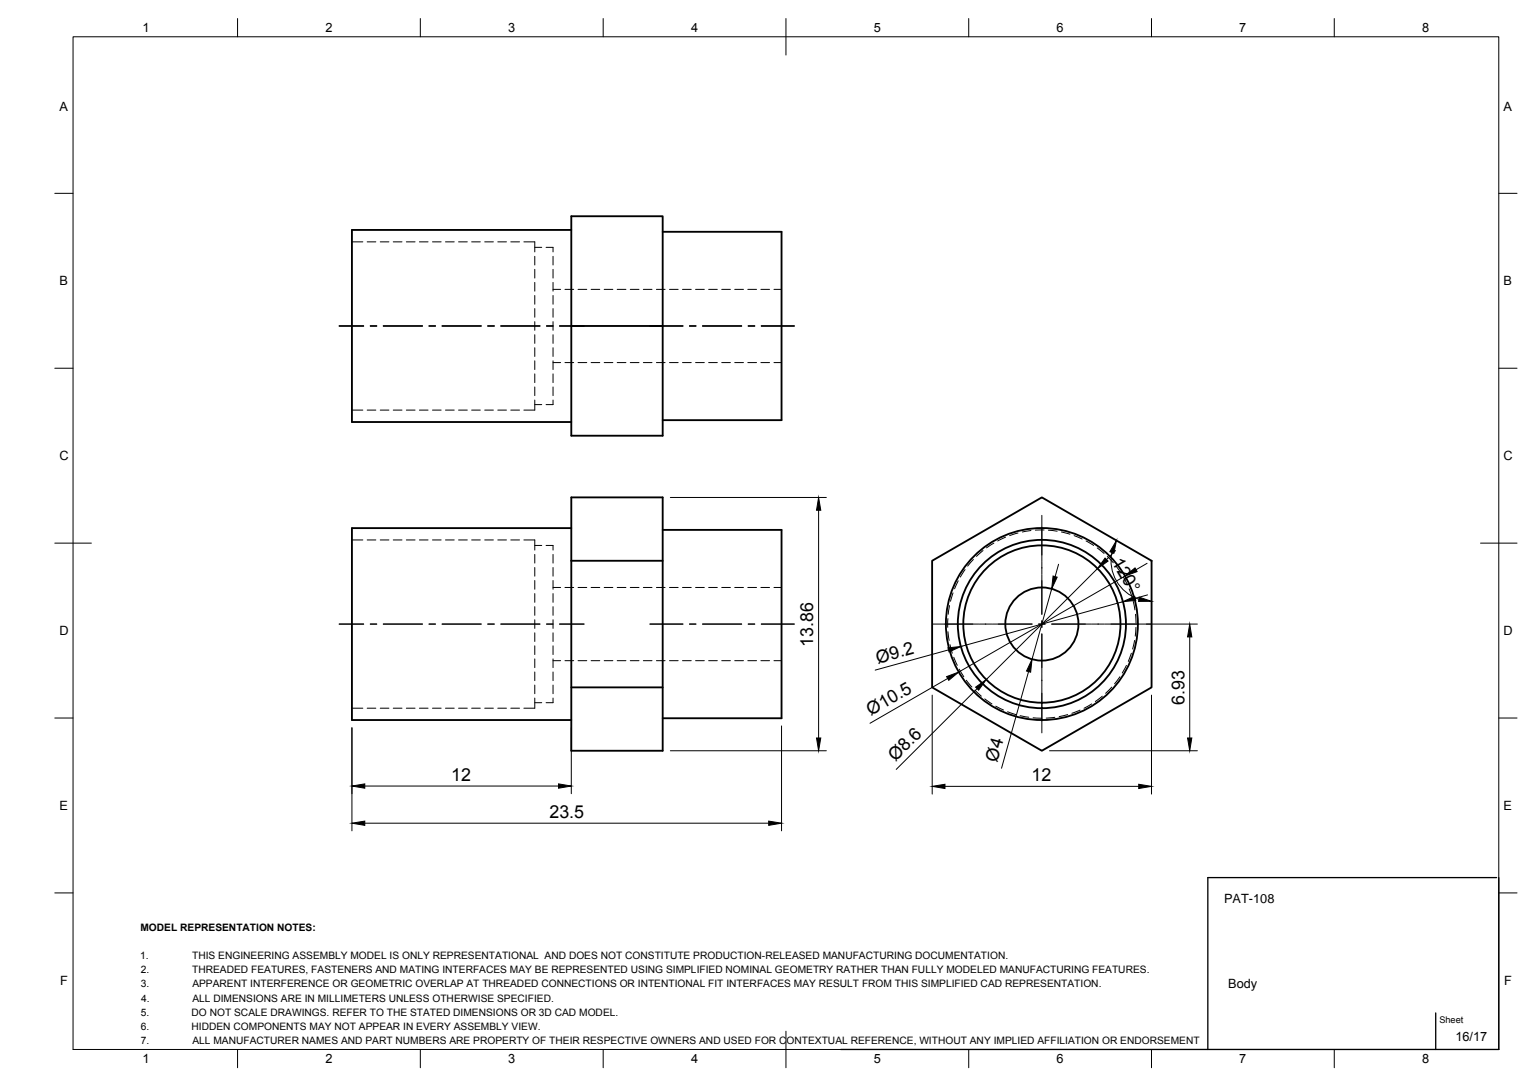
ISO-10303-21;
HEADER;
/* Generated by software containing ST-Developer
 * from STEP Tools, Inc. (www.steptools.com) 
 */

FILE_DESCRIPTION(
/* description */ ('Sub-base valve envelopes and connections'),
/* implementation_level */ '2;1');

FILE_NAME(
/* name */ 'Body.step',
/* time_stamp */ '2026-10-29T15:55:44-07:00',
/* author */ (''),
/* organization */ (''),
/* preprocessor_version */ 'ST-DEVELOPER v20.2',
/* originating_system */ 'Autodesk Translation Framework v15.17.0.0',
/* authorisation */ '');

FILE_SCHEMA (('AUTOMOTIVE_DESIGN { 1 0 10303 214 3 1 1 }'));
ENDSEC;

DATA;
#10=MECHANICAL_DESIGN_GEOMETRIC_PRESENTATION_REPRESENTATION('',(#128),#6113);
#104=SHAPE_REPRESENTATION_RELATIONSHIP('SRR','None',#6179,#116);
#116=ADVANCED_BREP_SHAPE_REPRESENTATION('',(#140),#6110);
#128=STYLED_ITEM('',(#6294),#140);
#140=MANIFOLD_SOLID_BREP('Body1',#3367);
#249=FACE_BOUND('',#853,.T.);
#250=FACE_BOUND('',#855,.T.);
#251=FACE_BOUND('',#857,.T.);
#252=FACE_BOUND('',#865,.T.);
#253=FACE_BOUND('',#868,.T.);
#254=FACE_BOUND('',#872,.T.);
#360=PLANE('',#3823);
#361=PLANE('',#3825);
#362=PLANE('',#3827);
#363=PLANE('',#3829);
#364=PLANE('',#3830);
#365=PLANE('',#3831);
#366=PLANE('',#3832);
#367=PLANE('',#3833);
#368=PLANE('',#3834);
#369=PLANE('',#3835);
#370=PLANE('',#3839);
#371=PLANE('',#3844);
#545=FACE_OUTER_BOUND('',#851,.T.);
#546=FACE_OUTER_BOUND('',#852,.T.);
#547=FACE_OUTER_BOUND('',#854,.T.);
#548=FACE_OUTER_BOUND('',#856,.T.);
#549=FACE_OUTER_BOUND('',#858,.T.);
#550=FACE_OUTER_BOUND('',#859,.T.);
#551=FACE_OUTER_BOUND('',#860,.T.);
#552=FACE_OUTER_BOUND('',#861,.T.);
#553=FACE_OUTER_BOUND('',#862,.T.);
#554=FACE_OUTER_BOUND('',#863,.T.);
#555=FACE_OUTER_BOUND('',#864,.T.);
#556=FACE_OUTER_BOUND('',#866,.T.);
#557=FACE_OUTER_BOUND('',#867,.T.);
#558=FACE_OUTER_BOUND('',#869,.T.);
#559=FACE_OUTER_BOUND('',#870,.T.);
#560=FACE_OUTER_BOUND('',#871,.T.);
#561=FACE_OUTER_BOUND('',#873,.T.);
#851=EDGE_LOOP('',(#2927,#2928,#2929,#2930));
#852=EDGE_LOOP('',(#2931));
#853=EDGE_LOOP('',(#2932));
#854=EDGE_LOOP('',(#2933,#2934,#2935,#2936,#2937,#2938));
#855=EDGE_LOOP('',(#2939));
#856=EDGE_LOOP('',(#2940,#2941,#2942,#2943,#2944,#2945));
#857=EDGE_LOOP('',(#2946));
#858=EDGE_LOOP('',(#2947,#2948,#2949,#2950));
#859=EDGE_LOOP('',(#2951,#2952,#2953,#2954));
#860=EDGE_LOOP('',(#2955,#2956,#2957,#2958));
#861=EDGE_LOOP('',(#2959,#2960,#2961,#2962));
#862=EDGE_LOOP('',(#2963,#2964,#2965,#2966));
#863=EDGE_LOOP('',(#2967,#2968,#2969,#2970));
#864=EDGE_LOOP('',(#2971));
#865=EDGE_LOOP('',(#2972));
#866=EDGE_LOOP('',(#2973,#2974,#2975,#2976));
#867=EDGE_LOOP('',(#2977));
#868=EDGE_LOOP('',(#2978));
#869=EDGE_LOOP('',(#2979,#2980,#2981,#2982));
#870=EDGE_LOOP('',(#2983,#2984,#2985,#2986));
#871=EDGE_LOOP('',(#2987));
#872=EDGE_LOOP('',(#2988));
#873=EDGE_LOOP('',(#2989,#2990,#2991,#2992));
#1085=LINE('',#5903,#1319);
#1086=LINE('',#5911,#1320);
#1087=LINE('',#5913,#1321);
#1088=LINE('',#5915,#1322);
#1089=LINE('',#5917,#1323);
#1090=LINE('',#5919,#1324);
#1091=LINE('',#5920,#1325);
#1092=LINE('',#5926,#1326);
#1093=LINE('',#5928,#1327);
#1094=LINE('',#5930,#1328);
#1095=LINE('',#5932,#1329);
#1096=LINE('',#5934,#1330);
#1097=LINE('',#5935,#1331);
#1098=LINE('',#5939,#1332);
#1099=LINE('',#5940,#1333);
#1100=LINE('',#5942,#1334);
#1101=LINE('',#5944,#1335);
#1102=LINE('',#5946,#1336);
#1103=LINE('',#5948,#1337);
#1104=LINE('',#5955,#1338);
#1105=LINE('',#5961,#1339);
#1106=LINE('',#5965,#1340);
#1107=LINE('',#5970,#1341);
#1319=VECTOR('',#4725,0.43);
#1320=VECTOR('',#4734,1.);
#1321=VECTOR('',#4735,1.);
#1322=VECTOR('',#4736,1.);
#1323=VECTOR('',#4737,1.);
#1324=VECTOR('',#4738,1.);
#1325=VECTOR('',#4739,1.);
#1326=VECTOR('',#4744,1.);
#1327=VECTOR('',#4745,1.);
#1328=VECTOR('',#4746,1.);
#1329=VECTOR('',#4747,1.);
#1330=VECTOR('',#4748,1.);
#1331=VECTOR('',#4749,1.);
#1332=VECTOR('',#4754,1.);
#1333=VECTOR('',#4755,1.);
#1334=VECTOR('',#4758,1.);
#1335=VECTOR('',#4761,1.);
#1336=VECTOR('',#4764,1.);
#1337=VECTOR('',#4767,1.);
#1338=VECTOR('',#4776,0.46);
#1339=VECTOR('',#4785,0.525);
#1340=VECTOR('',#4790,0.515);
#1341=VECTOR('',#4797,0.2);
#1513=CIRCLE('',#3821,0.43);
#1514=CIRCLE('',#3822,0.43);
#1515=CIRCLE('',#3824,0.2);
#1516=CIRCLE('',#3826,0.525);
#1517=CIRCLE('',#3828,0.515);
#1518=CIRCLE('',#3836,0.46);
#1519=CIRCLE('',#3838,0.46);
#1520=CIRCLE('',#3840,0.525);
#1521=CIRCLE('',#3843,0.515);
#1522=CIRCLE('',#3845,0.2);
#1767=VERTEX_POINT('',#5900);
#1768=VERTEX_POINT('',#5902);
#1769=VERTEX_POINT('',#5906);
#1770=VERTEX_POINT('',#5909);
#1771=VERTEX_POINT('',#5910);
#1772=VERTEX_POINT('',#5912);
#1773=VERTEX_POINT('',#5914);
#1774=VERTEX_POINT('',#5916);
#1775=VERTEX_POINT('',#5918);
#1776=VERTEX_POINT('',#5921);
#1777=VERTEX_POINT('',#5924);
#1778=VERTEX_POINT('',#5925);
#1779=VERTEX_POINT('',#5927);
#1780=VERTEX_POINT('',#5929);
#1781=VERTEX_POINT('',#5931);
#1782=VERTEX_POINT('',#5933);
#1783=VERTEX_POINT('',#5936);
#1784=VERTEX_POINT('',#5951);
#1785=VERTEX_POINT('',#5954);
#1786=VERTEX_POINT('',#5958);
#1787=VERTEX_POINT('',#5963);
#1788=VERTEX_POINT('',#5967);
#2161=EDGE_CURVE('',#1767,#1767,#1513,.T.);
#2162=EDGE_CURVE('',#1767,#1768,#1085,.T.);
#2163=EDGE_CURVE('',#1768,#1768,#1514,.T.);
#2164=EDGE_CURVE('',#1769,#1769,#1515,.T.);
#2165=EDGE_CURVE('',#1770,#1771,#1086,.T.);
#2166=EDGE_CURVE('',#1771,#1772,#1087,.T.);
#2167=EDGE_CURVE('',#1772,#1773,#1088,.T.);
#2168=EDGE_CURVE('',#1773,#1774,#1089,.T.);
#2169=EDGE_CURVE('',#1774,#1775,#1090,.T.);
#2170=EDGE_CURVE('',#1775,#1770,#1091,.T.);
#2171=EDGE_CURVE('',#1776,#1776,#1516,.T.);
#2172=EDGE_CURVE('',#1777,#1778,#1092,.T.);
#2173=EDGE_CURVE('',#1779,#1777,#1093,.T.);
#2174=EDGE_CURVE('',#1780,#1779,#1094,.T.);
#2175=EDGE_CURVE('',#1781,#1780,#1095,.T.);
#2176=EDGE_CURVE('',#1782,#1781,#1096,.T.);
#2177=EDGE_CURVE('',#1778,#1782,#1097,.T.);
#2178=EDGE_CURVE('',#1783,#1783,#1517,.T.);
#2179=EDGE_CURVE('',#1777,#1770,#1098,.T.);
#2180=EDGE_CURVE('',#1779,#1775,#1099,.T.);
#2181=EDGE_CURVE('',#1780,#1774,#1100,.T.);
#2182=EDGE_CURVE('',#1781,#1773,#1101,.T.);
#2183=EDGE_CURVE('',#1782,#1772,#1102,.T.);
#2184=EDGE_CURVE('',#1778,#1771,#1103,.T.);
#2185=EDGE_CURVE('',#1784,#1784,#1518,.T.);
#2186=EDGE_CURVE('',#1784,#1785,#1104,.T.);
#2187=EDGE_CURVE('',#1785,#1785,#1519,.T.);
#2188=EDGE_CURVE('',#1786,#1786,#1520,.T.);
#2189=EDGE_CURVE('',#1776,#1786,#1105,.T.);
#2190=EDGE_CURVE('',#1787,#1787,#1521,.T.);
#2191=EDGE_CURVE('',#1787,#1783,#1106,.T.);
#2192=EDGE_CURVE('',#1788,#1788,#1522,.T.);
#2193=EDGE_CURVE('',#1788,#1769,#1107,.T.);
#2927=ORIENTED_EDGE('',*,*,#2161,.F.);
#2928=ORIENTED_EDGE('',*,*,#2162,.T.);
#2929=ORIENTED_EDGE('',*,*,#2163,.F.);
#2930=ORIENTED_EDGE('',*,*,#2162,.F.);
#2931=ORIENTED_EDGE('',*,*,#2161,.T.);
#2932=ORIENTED_EDGE('',*,*,#2164,.F.);
#2933=ORIENTED_EDGE('',*,*,#2165,.T.);
#2934=ORIENTED_EDGE('',*,*,#2166,.T.);
#2935=ORIENTED_EDGE('',*,*,#2167,.T.);
#2936=ORIENTED_EDGE('',*,*,#2168,.T.);
#2937=ORIENTED_EDGE('',*,*,#2169,.T.);
#2938=ORIENTED_EDGE('',*,*,#2170,.T.);
#2939=ORIENTED_EDGE('',*,*,#2171,.T.);
#2940=ORIENTED_EDGE('',*,*,#2172,.F.);
#2941=ORIENTED_EDGE('',*,*,#2173,.F.);
#2942=ORIENTED_EDGE('',*,*,#2174,.F.);
#2943=ORIENTED_EDGE('',*,*,#2175,.F.);
#2944=ORIENTED_EDGE('',*,*,#2176,.F.);
#2945=ORIENTED_EDGE('',*,*,#2177,.F.);
#2946=ORIENTED_EDGE('',*,*,#2178,.F.);
#2947=ORIENTED_EDGE('',*,*,#2173,.T.);
#2948=ORIENTED_EDGE('',*,*,#2179,.T.);
#2949=ORIENTED_EDGE('',*,*,#2170,.F.);
#2950=ORIENTED_EDGE('',*,*,#2180,.F.);
#2951=ORIENTED_EDGE('',*,*,#2174,.T.);
#2952=ORIENTED_EDGE('',*,*,#2180,.T.);
#2953=ORIENTED_EDGE('',*,*,#2169,.F.);
#2954=ORIENTED_EDGE('',*,*,#2181,.F.);
#2955=ORIENTED_EDGE('',*,*,#2175,.T.);
#2956=ORIENTED_EDGE('',*,*,#2181,.T.);
#2957=ORIENTED_EDGE('',*,*,#2168,.F.);
#2958=ORIENTED_EDGE('',*,*,#2182,.F.);
#2959=ORIENTED_EDGE('',*,*,#2176,.T.);
#2960=ORIENTED_EDGE('',*,*,#2182,.T.);
#2961=ORIENTED_EDGE('',*,*,#2167,.F.);
#2962=ORIENTED_EDGE('',*,*,#2183,.F.);
#2963=ORIENTED_EDGE('',*,*,#2177,.T.);
#2964=ORIENTED_EDGE('',*,*,#2183,.T.);
#2965=ORIENTED_EDGE('',*,*,#2166,.F.);
#2966=ORIENTED_EDGE('',*,*,#2184,.F.);
#2967=ORIENTED_EDGE('',*,*,#2172,.T.);
#2968=ORIENTED_EDGE('',*,*,#2184,.T.);
#2969=ORIENTED_EDGE('',*,*,#2165,.F.);
#2970=ORIENTED_EDGE('',*,*,#2179,.F.);
#2971=ORIENTED_EDGE('',*,*,#2185,.F.);
#2972=ORIENTED_EDGE('',*,*,#2163,.T.);
#2973=ORIENTED_EDGE('',*,*,#2185,.T.);
#2974=ORIENTED_EDGE('',*,*,#2186,.T.);
#2975=ORIENTED_EDGE('',*,*,#2187,.F.);
#2976=ORIENTED_EDGE('',*,*,#2186,.F.);
#2977=ORIENTED_EDGE('',*,*,#2188,.F.);
#2978=ORIENTED_EDGE('',*,*,#2187,.T.);
#2979=ORIENTED_EDGE('',*,*,#2171,.F.);
#2980=ORIENTED_EDGE('',*,*,#2189,.T.);
#2981=ORIENTED_EDGE('',*,*,#2188,.T.);
#2982=ORIENTED_EDGE('',*,*,#2189,.F.);
#2983=ORIENTED_EDGE('',*,*,#2190,.F.);
#2984=ORIENTED_EDGE('',*,*,#2191,.T.);
#2985=ORIENTED_EDGE('',*,*,#2178,.T.);
#2986=ORIENTED_EDGE('',*,*,#2191,.F.);
#2987=ORIENTED_EDGE('',*,*,#2190,.T.);
#2988=ORIENTED_EDGE('',*,*,#2192,.F.);
#2989=ORIENTED_EDGE('',*,*,#2192,.T.);
#2990=ORIENTED_EDGE('',*,*,#2193,.T.);
#2991=ORIENTED_EDGE('',*,*,#2164,.T.);
#2992=ORIENTED_EDGE('',*,*,#2193,.F.);
#3149=CYLINDRICAL_SURFACE('',#3820,0.43);
#3150=CYLINDRICAL_SURFACE('',#3837,0.46);
#3151=CYLINDRICAL_SURFACE('',#3841,0.525);
#3152=CYLINDRICAL_SURFACE('',#3842,0.515);
#3153=CYLINDRICAL_SURFACE('',#3846,0.2);
#3318=ADVANCED_FACE('',(#545),#3149,.F.);
#3319=ADVANCED_FACE('',(#546,#249),#360,.T.);
#3320=ADVANCED_FACE('',(#547,#250),#361,.T.);
#3321=ADVANCED_FACE('',(#548,#251),#362,.F.);
#3322=ADVANCED_FACE('',(#549),#363,.T.);
#3323=ADVANCED_FACE('',(#550),#364,.T.);
#3324=ADVANCED_FACE('',(#551),#365,.T.);
#3325=ADVANCED_FACE('',(#552),#366,.T.);
#3326=ADVANCED_FACE('',(#553),#367,.T.);
#3327=ADVANCED_FACE('',(#554),#368,.T.);
#3328=ADVANCED_FACE('',(#555,#252),#369,.T.);
#3329=ADVANCED_FACE('',(#556),#3150,.F.);
#3330=ADVANCED_FACE('',(#557,#253),#370,.T.);
#3331=ADVANCED_FACE('',(#558),#3151,.T.);
#3332=ADVANCED_FACE('',(#559),#3152,.T.);
#3333=ADVANCED_FACE('',(#560,#254),#371,.T.);
#3334=ADVANCED_FACE('',(#561),#3153,.F.);
#3367=CLOSED_SHELL('',(#3318,#3319,#3320,#3321,#3322,#3323,#3324,#3325,
#3326,#3327,#3328,#3329,#3330,#3331,#3332,#3333,#3334));
#3819=AXIS2_PLACEMENT_3D('',#5898,#4719,#4720);
#3820=AXIS2_PLACEMENT_3D('',#5899,#4721,#4722);
#3821=AXIS2_PLACEMENT_3D('',#5901,#4723,#4724);
#3822=AXIS2_PLACEMENT_3D('',#5904,#4726,#4727);
#3823=AXIS2_PLACEMENT_3D('',#5905,#4728,#4729);
#3824=AXIS2_PLACEMENT_3D('',#5907,#4730,#4731);
#3825=AXIS2_PLACEMENT_3D('',#5908,#4732,#4733);
#3826=AXIS2_PLACEMENT_3D('',#5922,#4740,#4741);
#3827=AXIS2_PLACEMENT_3D('',#5923,#4742,#4743);
#3828=AXIS2_PLACEMENT_3D('',#5937,#4750,#4751);
#3829=AXIS2_PLACEMENT_3D('',#5938,#4752,#4753);
#3830=AXIS2_PLACEMENT_3D('',#5941,#4756,#4757);
#3831=AXIS2_PLACEMENT_3D('',#5943,#4759,#4760);
#3832=AXIS2_PLACEMENT_3D('',#5945,#4762,#4763);
#3833=AXIS2_PLACEMENT_3D('',#5947,#4765,#4766);
#3834=AXIS2_PLACEMENT_3D('',#5949,#4768,#4769);
#3835=AXIS2_PLACEMENT_3D('',#5950,#4770,#4771);
#3836=AXIS2_PLACEMENT_3D('',#5952,#4772,#4773);
#3837=AXIS2_PLACEMENT_3D('',#5953,#4774,#4775);
#3838=AXIS2_PLACEMENT_3D('',#5956,#4777,#4778);
#3839=AXIS2_PLACEMENT_3D('',#5957,#4779,#4780);
#3840=AXIS2_PLACEMENT_3D('',#5959,#4781,#4782);
#3841=AXIS2_PLACEMENT_3D('',#5960,#4783,#4784);
#3842=AXIS2_PLACEMENT_3D('',#5962,#4786,#4787);
#3843=AXIS2_PLACEMENT_3D('',#5964,#4788,#4789);
#3844=AXIS2_PLACEMENT_3D('',#5966,#4791,#4792);
#3845=AXIS2_PLACEMENT_3D('',#5968,#4793,#4794);
#3846=AXIS2_PLACEMENT_3D('',#5969,#4795,#4796);
#4719=DIRECTION('axis',(0.,0.,1.));
#4720=DIRECTION('refdir',(1.,0.,0.));
#4721=DIRECTION('center_axis',(0.,1.,0.));
#4722=DIRECTION('ref_axis',(1.,0.,0.));
#4723=DIRECTION('center_axis',(0.,1.,0.));
#4724=DIRECTION('ref_axis',(1.,0.,0.));
#4725=DIRECTION('',(0.,1.,0.));
#4726=DIRECTION('center_axis',(0.,-1.,0.));
#4727=DIRECTION('ref_axis',(1.,0.,0.));
#4728=DIRECTION('center_axis',(0.,1.,0.));
#4729=DIRECTION('ref_axis',(1.,0.,0.));
#4730=DIRECTION('center_axis',(0.,1.,0.));
#4731=DIRECTION('ref_axis',(1.,0.,0.));
#4732=DIRECTION('center_axis',(0.,1.,0.));
#4733=DIRECTION('ref_axis',(1.,0.,0.));
#4734=DIRECTION('',(0.5,0.,-0.866025403784439));
#4735=DIRECTION('',(-0.5,0.,-0.866025403784439));
#4736=DIRECTION('',(-1.,0.,-1.60246890531964E-16));
#4737=DIRECTION('',(-0.5,0.,0.866025403784439));
#4738=DIRECTION('',(0.5,0.,0.866025403784439));
#4739=DIRECTION('',(1.,0.,1.60246890531964E-16));
#4740=DIRECTION('center_axis',(0.,-1.,0.));
#4741=DIRECTION('ref_axis',(1.,0.,0.));
#4742=DIRECTION('center_axis',(0.,1.,0.));
#4743=DIRECTION('ref_axis',(1.,0.,0.));
#4744=DIRECTION('',(0.5,0.,-0.866025403784439));
#4745=DIRECTION('',(1.,0.,1.60246890531964E-16));
#4746=DIRECTION('',(0.5,0.,0.866025403784439));
#4747=DIRECTION('',(-0.5,0.,0.866025403784439));
#4748=DIRECTION('',(-1.,0.,-1.60246890531964E-16));
#4749=DIRECTION('',(-0.5,0.,-0.866025403784439));
#4750=DIRECTION('center_axis',(0.,-1.,0.));
#4751=DIRECTION('ref_axis',(1.,0.,0.));
#4752=DIRECTION('center_axis',(-1.60246890531964E-16,0.,1.));
#4753=DIRECTION('ref_axis',(1.,0.,1.60246890531964E-16));
#4754=DIRECTION('',(0.,1.,0.));
#4755=DIRECTION('',(0.,1.,0.));
#4756=DIRECTION('center_axis',(-0.866025403784439,0.,0.5));
#4757=DIRECTION('ref_axis',(0.5,0.,0.866025403784439));
#4758=DIRECTION('',(0.,1.,0.));
#4759=DIRECTION('center_axis',(-0.866025403784439,0.,-0.5));
#4760=DIRECTION('ref_axis',(-0.5,0.,0.866025403784439));
#4761=DIRECTION('',(0.,1.,0.));
#4762=DIRECTION('center_axis',(1.60246890531964E-16,0.,-1.));
#4763=DIRECTION('ref_axis',(-1.,0.,-1.60246890531964E-16));
#4764=DIRECTION('',(0.,1.,0.));
#4765=DIRECTION('center_axis',(0.866025403784439,0.,-0.5));
#4766=DIRECTION('ref_axis',(-0.5,0.,-0.866025403784439));
#4767=DIRECTION('',(0.,1.,0.));
#4768=DIRECTION('center_axis',(0.866025403784439,0.,0.5));
#4769=DIRECTION('ref_axis',(0.5,0.,-0.866025403784439));
#4770=DIRECTION('center_axis',(0.,1.,0.));
#4771=DIRECTION('ref_axis',(0.,0.,1.));
#4772=DIRECTION('center_axis',(0.,-1.,0.));
#4773=DIRECTION('ref_axis',(1.,0.,0.));
#4774=DIRECTION('center_axis',(0.,-1.,0.));
#4775=DIRECTION('ref_axis',(1.,0.,0.));
#4776=DIRECTION('',(0.,1.,0.));
#4777=DIRECTION('center_axis',(0.,-1.,0.));
#4778=DIRECTION('ref_axis',(1.,0.,0.));
#4779=DIRECTION('center_axis',(0.,1.,0.));
#4780=DIRECTION('ref_axis',(0.,0.,1.));
#4781=DIRECTION('center_axis',(0.,-1.,0.));
#4782=DIRECTION('ref_axis',(1.,0.,0.));
#4783=DIRECTION('center_axis',(0.,-1.,0.));
#4784=DIRECTION('ref_axis',(1.,0.,0.));
#4785=DIRECTION('',(0.,1.,0.));
#4786=DIRECTION('center_axis',(0.,-1.,0.));
#4787=DIRECTION('ref_axis',(1.,0.,0.));
#4788=DIRECTION('center_axis',(0.,-1.,0.));
#4789=DIRECTION('ref_axis',(1.,0.,0.));
#4790=DIRECTION('',(0.,1.,0.));
#4791=DIRECTION('center_axis',(0.,-1.,0.));
#4792=DIRECTION('ref_axis',(0.,0.,-1.));
#4793=DIRECTION('center_axis',(0.,-1.,0.));
#4794=DIRECTION('ref_axis',(1.,0.,0.));
#4795=DIRECTION('center_axis',(0.,-1.,0.));
#4796=DIRECTION('ref_axis',(1.,0.,0.));
#4797=DIRECTION('',(0.,1.,0.));
#5898=CARTESIAN_POINT('',(0.,0.,0.));
#5899=CARTESIAN_POINT('Origin',(0.,0.6,0.));
#5900=CARTESIAN_POINT('',(-0.43,0.6,5.26598123633362E-17));
#5901=CARTESIAN_POINT('Origin',(0.,0.6,0.));
#5902=CARTESIAN_POINT('',(-0.43,0.7,-5.26598123633362E-17));
#5903=CARTESIAN_POINT('',(-0.43,0.6,5.26598123633362E-17));
#5904=CARTESIAN_POINT('Origin',(0.,0.7,0.));
#5905=CARTESIAN_POINT('Origin',(0.,0.6,0.));
#5906=CARTESIAN_POINT('',(-0.2,0.6,2.44929359829471E-17));
#5907=CARTESIAN_POINT('Origin',(0.,0.6,0.));
#5908=CARTESIAN_POINT('Origin',(0.,0.5,-1.11022302462516E-16));
#5909=CARTESIAN_POINT('',(0.346410161513776,0.5,0.6));
#5910=CARTESIAN_POINT('',(0.692820323027551,0.5,0.));
#5911=CARTESIAN_POINT('',(0.346410161513776,0.5,0.6));
#5912=CARTESIAN_POINT('',(0.346410161513776,0.5,-0.6));
#5913=CARTESIAN_POINT('',(0.692820323027551,0.5,0.));
#5914=CARTESIAN_POINT('',(-0.346410161513775,0.5,-0.6));
#5915=CARTESIAN_POINT('',(0.346410161513776,0.5,-0.6));
#5916=CARTESIAN_POINT('',(-0.692820323027551,0.5,-8.48460190979926E-17));
#5917=CARTESIAN_POINT('',(-0.346410161513775,0.5,-0.6));
#5918=CARTESIAN_POINT('',(-0.346410161513776,0.5,0.6));
#5919=CARTESIAN_POINT('',(-0.692820323027551,0.5,-8.48460190979926E-17));
#5920=CARTESIAN_POINT('',(-0.346410161513776,0.5,0.6));
#5921=CARTESIAN_POINT('',(-0.525,0.5,-6.4293956955236E-17));
#5922=CARTESIAN_POINT('Origin',(0.,0.5,0.));
#5923=CARTESIAN_POINT('Origin',(0.,0.,-1.11022302462516E-16));
#5924=CARTESIAN_POINT('',(0.346410161513776,0.,0.6));
#5925=CARTESIAN_POINT('',(0.692820323027551,0.,0.));
#5926=CARTESIAN_POINT('',(0.346410161513776,0.,0.6));
#5927=CARTESIAN_POINT('',(-0.346410161513776,0.,0.6));
#5928=CARTESIAN_POINT('',(-0.346410161513776,0.,0.6));
#5929=CARTESIAN_POINT('',(-0.692820323027551,0.,-8.48460190979926E-17));
#5930=CARTESIAN_POINT('',(-0.692820323027551,0.,-8.48460190979926E-17));
#5931=CARTESIAN_POINT('',(-0.346410161513775,0.,-0.6));
#5932=CARTESIAN_POINT('',(-0.346410161513775,0.,-0.6));
#5933=CARTESIAN_POINT('',(0.346410161513776,0.,-0.6));
#5934=CARTESIAN_POINT('',(0.346410161513776,0.,-0.6));
#5935=CARTESIAN_POINT('',(0.692820323027551,0.,0.));
#5936=CARTESIAN_POINT('',(-0.515,0.,-6.30693101560887E-17));
#5937=CARTESIAN_POINT('Origin',(0.,0.,0.));
#5938=CARTESIAN_POINT('Origin',(-0.346410161513776,0.,0.6));
#5939=CARTESIAN_POINT('',(0.346410161513776,0.,0.6));
#5940=CARTESIAN_POINT('',(-0.346410161513776,0.,0.6));
#5941=CARTESIAN_POINT('Origin',(-0.692820323027551,0.,-8.48460190979926E-17));
#5942=CARTESIAN_POINT('',(-0.692820323027551,0.,-8.48460190979926E-17));
#5943=CARTESIAN_POINT('Origin',(-0.346410161513775,0.,-0.6));
#5944=CARTESIAN_POINT('',(-0.346410161513775,0.,-0.6));
#5945=CARTESIAN_POINT('Origin',(0.346410161513776,0.,-0.6));
#5946=CARTESIAN_POINT('',(0.346410161513776,0.,-0.6));
#5947=CARTESIAN_POINT('Origin',(0.692820323027551,0.,0.));
#5948=CARTESIAN_POINT('',(0.692820323027551,0.,0.));
#5949=CARTESIAN_POINT('Origin',(0.346410161513776,0.,0.6));
#5950=CARTESIAN_POINT('Origin',(0.46,0.7,0.));
#5951=CARTESIAN_POINT('',(-0.46,0.7,-5.63337527607782E-17));
#5952=CARTESIAN_POINT('Origin',(0.,0.7,0.));
#5953=CARTESIAN_POINT('Origin',(0.,1.2,0.));
#5954=CARTESIAN_POINT('',(-0.46,1.7,-5.63337527607782E-17));
#5955=CARTESIAN_POINT('',(-0.46,1.2,-5.63337527607782E-17));
#5956=CARTESIAN_POINT('Origin',(0.,1.7,0.));
#5957=CARTESIAN_POINT('Origin',(0.525,1.7,0.));
#5958=CARTESIAN_POINT('',(-0.525,1.7,-6.4293956955236E-17));
#5959=CARTESIAN_POINT('Origin',(0.,1.7,0.));
#5960=CARTESIAN_POINT('Origin',(0.,1.1,0.));
#5961=CARTESIAN_POINT('',(-0.525,1.1,-6.4293956955236E-17));
#5962=CARTESIAN_POINT('Origin',(0.,-0.325,0.));
#5963=CARTESIAN_POINT('',(-0.515,-0.65,-6.30693101560887E-17));
#5964=CARTESIAN_POINT('Origin',(0.,-0.65,0.));
#5965=CARTESIAN_POINT('',(-0.515,-0.325,-6.30693101560887E-17));
#5966=CARTESIAN_POINT('Origin',(0.2,-0.65,0.));
#5967=CARTESIAN_POINT('',(-0.2,-0.65,-2.44929359829471E-17));
#5968=CARTESIAN_POINT('Origin',(0.,-0.65,0.));
#5969=CARTESIAN_POINT('Origin',(0.,0.0249999999999999,0.));
#5970=CARTESIAN_POINT('',(-0.2,0.0249999999999999,-2.44929359829471E-17));
#6094=UNCERTAINTY_MEASURE_WITH_UNIT(LENGTH_MEASURE(0.001),#6114,
'DISTANCE_ACCURACY_VALUE',
'Maximum model space distance between geometric entities at asserted c
onnectivities');
#6097=UNCERTAINTY_MEASURE_WITH_UNIT(LENGTH_MEASURE(0.001),#6114,
'DISTANCE_ACCURACY_VALUE',
'Maximum model space distance between geometric entities at asserted c
onnectivities');
#6110=(
GEOMETRIC_REPRESENTATION_CONTEXT(3)
GLOBAL_UNCERTAINTY_ASSIGNED_CONTEXT((#6094))
GLOBAL_UNIT_ASSIGNED_CONTEXT((#6114,#6116,#6117))
REPRESENTATION_CONTEXT('','3D')
);
#6113=(
GEOMETRIC_REPRESENTATION_CONTEXT(3)
GLOBAL_UNCERTAINTY_ASSIGNED_CONTEXT((#6097))
GLOBAL_UNIT_ASSIGNED_CONTEXT((#6114,#6116,#6117))
REPRESENTATION_CONTEXT('','3D')
);
#6114=(
LENGTH_UNIT()
NAMED_UNIT(*)
SI_UNIT(.CENTI.,.METRE.)
);
#6116=(
NAMED_UNIT(*)
PLANE_ANGLE_UNIT()
SI_UNIT($,.RADIAN.)
);
#6117=(
NAMED_UNIT(*)
SI_UNIT($,.STERADIAN.)
SOLID_ANGLE_UNIT()
);
#6130=SHAPE_DEFINITION_REPRESENTATION(#6145,#6179);
#6145=PRODUCT_DEFINITION_SHAPE('',$,#6195);
#6179=SHAPE_REPRESENTATION('',(#3819),#6110);
#6182=PRODUCT_DEFINITION_CONTEXT('part definition',#6229,'design');
#6195=PRODUCT_DEFINITION('Body','Body',#6210,#6182);
#6210=PRODUCT_DEFINITION_FORMATION('',$,#6243);
#6229=APPLICATION_CONTEXT(
'Core Data for Automotive Mechanical Design Process');
#6230=PRODUCT_CONTEXT('part definition',#6229,'mechanical');
#6243=PRODUCT('Body','Body','Body',(#6230));
#6288=COLOUR_RGB('Dark Blue',0.08,0.2,0.34);
#6289=FILL_AREA_STYLE_COLOUR('',#6288);
#6290=FILL_AREA_STYLE('',(#6289));
#6291=SURFACE_STYLE_FILL_AREA(#6290);
#6292=SURFACE_SIDE_STYLE('',(#6291));
#6293=SURFACE_STYLE_USAGE(.BOTH.,#6292);
#6294=PRESENTATION_STYLE_ASSIGNMENT((#6293));
ENDSEC;
END-ISO-10303-21;
